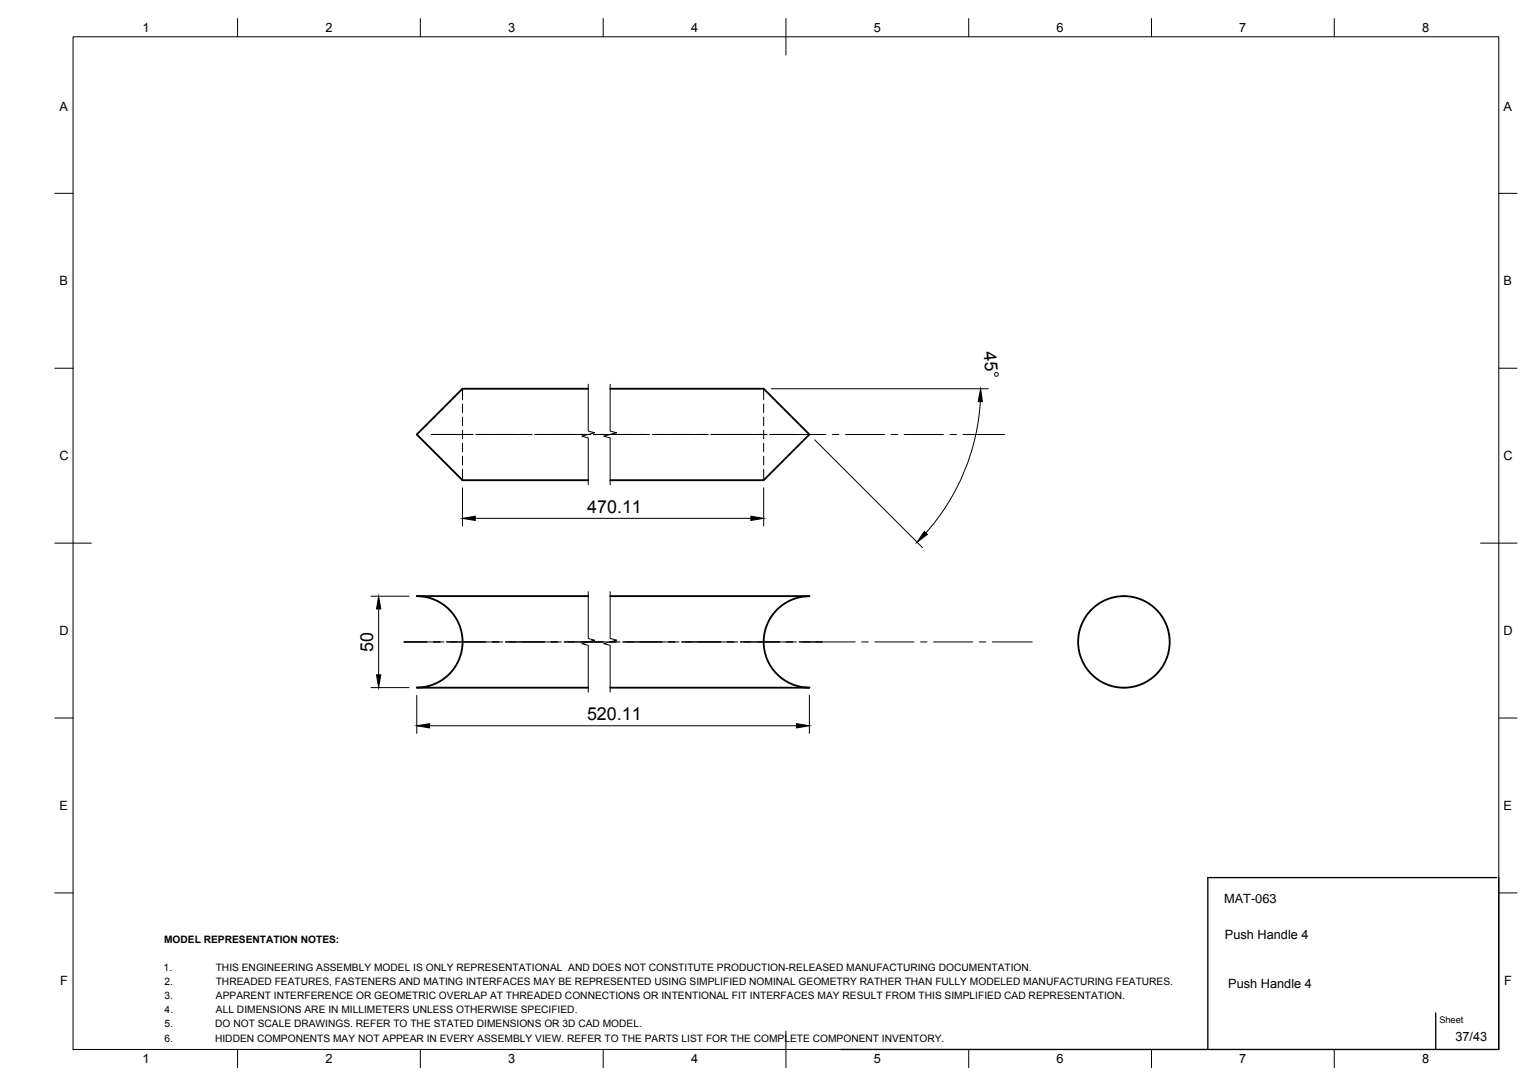
ISO-10303-21;
HEADER;
/* Generated by software containing ST-Developer
 * from STEP Tools, Inc. (www.steptools.com) 
 */

FILE_DESCRIPTION(
/* description */ (''),
/* implementation_level */ '2;1');

FILE_NAME(
/* name */ 'Push Handle 4.step',
/* time_stamp */ '2026-10-24T09:43:01-07:00',
/* author */ (''),
/* organization */ (''),
/* preprocessor_version */ 'ST-DEVELOPER v20.2',
/* originating_system */ 'Autodesk Translation Framework v15.15.0.0',
/* authorisation */ '');

FILE_SCHEMA (('AUTOMOTIVE_DESIGN { 1 0 10303 214 3 1 1 }'));
ENDSEC;

DATA;
#10=MECHANICAL_DESIGN_GEOMETRIC_PRESENTATION_REPRESENTATION('',(#300),#11112);
#15=ELLIPSE('',#7169,0.035355338987388,0.0249999999491312);
#16=ELLIPSE('',#7170,0.0353553389873879,0.0249999999491312);
#17=ELLIPSE('',#7172,0.0353553389873867,0.0249999999491303);
#18=ELLIPSE('',#7173,0.0353553389873867,0.0249999999491303);
#234=SHAPE_REPRESENTATION_RELATIONSHIP('SRR','None',#11260,#267);
#267=ADVANCED_BREP_SHAPE_REPRESENTATION('',(#333),#11105);
#300=STYLED_ITEM('',(#11426),#333);
#333=MANIFOLD_SOLID_BREP('Push Handle 4',#6037);
#1007=FACE_OUTER_BOUND('',#1513,.T.);
#1008=FACE_OUTER_BOUND('',#1514,.T.);
#1009=FACE_OUTER_BOUND('',#1515,.T.);
#1513=EDGE_LOOP('',(#5393,#5394));
#1514=EDGE_LOOP('',(#5395,#5396,#5397,#5398,#5399,#5400));
#1515=EDGE_LOOP('',(#5401,#5402));
#1896=LINE('',#10893,#2255);
#2255=VECTOR('',#9128,0.0249999998982604);
#3144=VERTEX_POINT('',#10887);
#3145=VERTEX_POINT('',#10888);
#3146=VERTEX_POINT('',#10892);
#3147=VERTEX_POINT('',#10894);
#3900=EDGE_CURVE('',#3144,#3145,#15,.T.);
#3901=EDGE_CURVE('',#3145,#3144,#16,.F.);
#3902=EDGE_CURVE('',#3144,#3146,#1896,.T.);
#3903=EDGE_CURVE('',#3146,#3147,#17,.T.);
#3904=EDGE_CURVE('',#3147,#3146,#18,.F.);
#5393=ORIENTED_EDGE('',*,*,#3900,.F.);
#5394=ORIENTED_EDGE('',*,*,#3901,.F.);
#5395=ORIENTED_EDGE('',*,*,#3901,.T.);
#5396=ORIENTED_EDGE('',*,*,#3902,.T.);
#5397=ORIENTED_EDGE('',*,*,#3903,.T.);
#5398=ORIENTED_EDGE('',*,*,#3904,.T.);
#5399=ORIENTED_EDGE('',*,*,#3902,.F.);
#5400=ORIENTED_EDGE('',*,*,#3900,.T.);
#5401=ORIENTED_EDGE('',*,*,#3903,.F.);
#5402=ORIENTED_EDGE('',*,*,#3904,.F.);
#5629=CYLINDRICAL_SURFACE('',#7168,0.0250000000000019);
#5630=CYLINDRICAL_SURFACE('',#7171,0.0249999998982604);
#5631=CYLINDRICAL_SURFACE('',#7174,0.025);
#5980=ADVANCED_FACE('',(#1007),#5629,.F.);
#5981=ADVANCED_FACE('',(#1008),#5630,.T.);
#5982=ADVANCED_FACE('',(#1009),#5631,.F.);
#6037=CLOSED_SHELL('',(#5980,#5981,#5982));
#7167=AXIS2_PLACEMENT_3D('',#10885,#9118,#9119);
#7168=AXIS2_PLACEMENT_3D('',#10886,#9120,#9121);
#7169=AXIS2_PLACEMENT_3D('',#10889,#9122,#9123);
#7170=AXIS2_PLACEMENT_3D('',#10890,#9124,#9125);
#7171=AXIS2_PLACEMENT_3D('',#10891,#9126,#9127);
#7172=AXIS2_PLACEMENT_3D('',#10895,#9129,#9130);
#7173=AXIS2_PLACEMENT_3D('',#10896,#9131,#9132);
#7174=AXIS2_PLACEMENT_3D('',#10897,#9133,#9134);
#9118=DIRECTION('axis',(0.,0.,1.));
#9119=DIRECTION('refdir',(1.,0.,0.));
#9120=DIRECTION('center_axis',(-1.,0.,2.22044604925031E-15));
#9121=DIRECTION('ref_axis',(-1.46909515046131E-15,0.749837855248542,-0.661621637218937));
#9122=DIRECTION('center_axis',(-0.707106781186548,0.530215432236494,-0.467837146257399));
#9123=DIRECTION('ref_axis',(-0.707106781186547,-0.530215432236493,0.467837146257402));
#9124=DIRECTION('center_axis',(-0.707106781186547,-0.530215432236493,0.467837146257402));
#9125=DIRECTION('ref_axis',(-0.707106781186548,0.530215432236494,-0.467837146257399));
#9126=DIRECTION('center_axis',(0.,-0.749837855248362,0.661621637219141));
#9127=DIRECTION('ref_axis',(0.,-0.661621637219141,-0.749837855248362));
#9128=DIRECTION('',(0.,0.749837855248362,-0.661621637219141));
#9129=DIRECTION('center_axis',(0.707106781186548,-0.530215432236494,0.4678371462574));
#9130=DIRECTION('ref_axis',(0.707106781186547,0.530215432236494,-0.4678371462574));
#9131=DIRECTION('center_axis',(0.707106781186548,0.530215432236494,-0.4678371462574));
#9132=DIRECTION('ref_axis',(0.707106781186547,-0.530215432236494,0.4678371462574));
#9133=DIRECTION('center_axis',(1.,0.,0.));
#9134=DIRECTION('ref_axis',(0.,-0.74983785524939,0.661621637217976));
#10885=CARTESIAN_POINT('',(0.,0.,0.));
#10886=CARTESIAN_POINT('Origin',(0.560710678,0.3,-0.955882353));
#10887=CARTESIAN_POINT('',(-0.30000000000004,0.316540540958999,-0.937136406587632));
#10888=CARTESIAN_POINT('',(-0.300000000000018,0.283459459165358,-0.974628299273766));
#10889=CARTESIAN_POINT('Origin',(-0.3,0.300000000061598,-0.955882352930187));
#10890=CARTESIAN_POINT('Origin',(-0.3,0.300000000061598,-0.955882352930187));
#10891=CARTESIAN_POINT('Origin',(-0.3,0.716460202,-1.323347237));
#10892=CARTESIAN_POINT('',(-0.300000000000012,0.70654054091276,-1.28125405363744));
#10893=CARTESIAN_POINT('',(-0.3,0.733000742863165,-1.30460129069508));
#10894=CARTESIAN_POINT('',(-0.300000000000004,0.673459459119238,-1.31874594632367));
#10895=CARTESIAN_POINT('Origin',(-0.3,0.690000000016651,-1.29999999998113));
#10896=CARTESIAN_POINT('Origin',(-0.3,0.690000000016651,-1.29999999998113));
#10897=CARTESIAN_POINT('Origin',(-0.35,0.69,-1.3));
#11066=UNCERTAINTY_MEASURE_WITH_UNIT(LENGTH_MEASURE(1.E-5),#11113,
'DISTANCE_ACCURACY_VALUE',
'Maximum model space distance between geometric entities at asserted c
onnectivities');
#11073=UNCERTAINTY_MEASURE_WITH_UNIT(LENGTH_MEASURE(1.E-5),#11113,
'DISTANCE_ACCURACY_VALUE',
'Maximum model space distance between geometric entities at asserted c
onnectivities');
#11105=(
GEOMETRIC_REPRESENTATION_CONTEXT(3)
GLOBAL_UNCERTAINTY_ASSIGNED_CONTEXT((#11066))
GLOBAL_UNIT_ASSIGNED_CONTEXT((#11113,#11114,#11115))
REPRESENTATION_CONTEXT('','3D')
);
#11112=(
GEOMETRIC_REPRESENTATION_CONTEXT(3)
GLOBAL_UNCERTAINTY_ASSIGNED_CONTEXT((#11073))
GLOBAL_UNIT_ASSIGNED_CONTEXT((#11113,#11114,#11115))
REPRESENTATION_CONTEXT('','3D')
);
#11113=(
LENGTH_UNIT()
NAMED_UNIT(*)
SI_UNIT($,.METRE.)
);
#11114=(
NAMED_UNIT(*)
PLANE_ANGLE_UNIT()
SI_UNIT($,.RADIAN.)
);
#11115=(
NAMED_UNIT(*)
SI_UNIT($,.STERADIAN.)
SOLID_ANGLE_UNIT()
);
#11147=SHAPE_DEFINITION_REPRESENTATION(#11198,#11260);
#11198=PRODUCT_DEFINITION_SHAPE('',$,#11299);
#11260=SHAPE_REPRESENTATION('',(#7167),#11105);
#11267=PRODUCT_DEFINITION_CONTEXT('part definition',#11383,'design');
#11299=PRODUCT_DEFINITION('Push Handle 4','Push Handle 4',#11337,#11267);
#11337=PRODUCT_DEFINITION_FORMATION('',$,#11416);
#11383=APPLICATION_CONTEXT(
'Core Data for Automotive Mechanical Design Process');
#11384=PRODUCT_CONTEXT('part definition',#11383,'mechanical');
#11416=PRODUCT('Push Handle 4','Push Handle 4',
'back_push__ DE     2873',(#11384));
#11426=PRESENTATION_STYLE_ASSIGNMENT((#11430));
#11430=SURFACE_STYLE_USAGE(.BOTH.,#11434);
#11434=SURFACE_SIDE_STYLE('',(#11438));
#11438=SURFACE_STYLE_FILL_AREA(#11442);
#11442=FILL_AREA_STYLE('Opaque(202,209,238)',(#11446));
#11446=FILL_AREA_STYLE_COLOUR('Opaque(202,209,238)',#11450);
#11450=COLOUR_RGB('Opaque(202,209,238)',0.792156862745098,0.819607843137255,
0.933333333333333);
ENDSEC;
END-ISO-10303-21;
